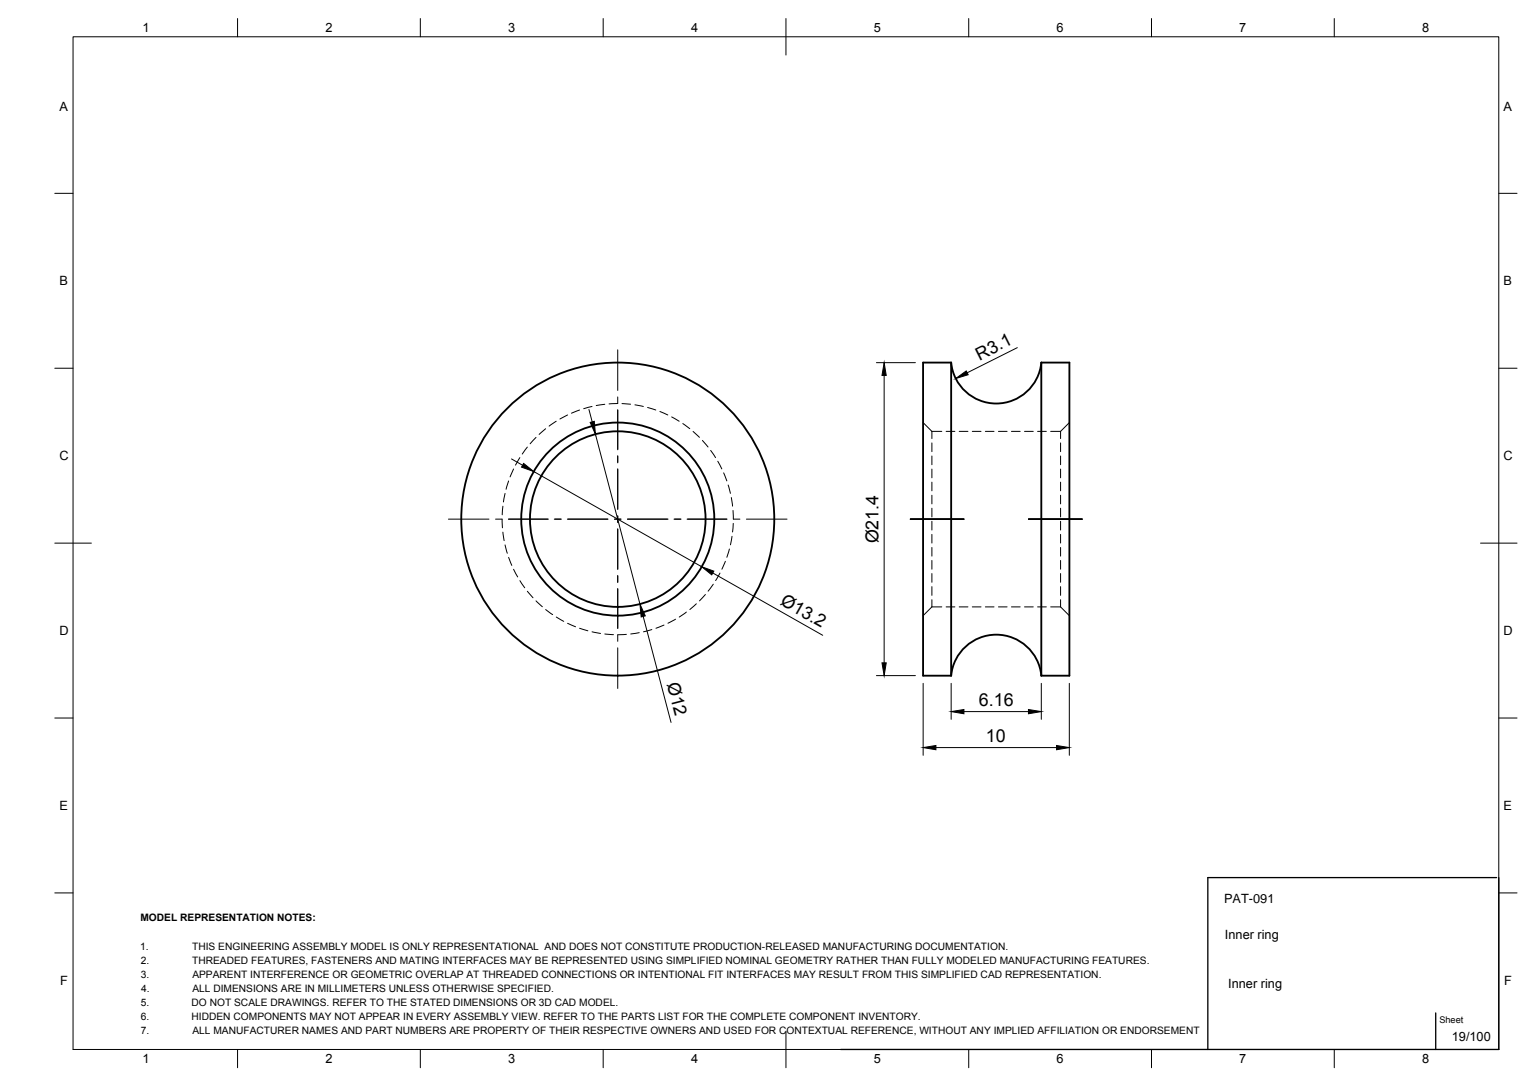
ISO-10303-21;
HEADER;
/* Generated by software containing ST-Developer
 * from STEP Tools, Inc. (www.steptools.com) 
 */

FILE_DESCRIPTION(
/* description */ ('PAT-091'),
/* implementation_level */ '2;1');

FILE_NAME(
/* name */ 'Inner ring.step',
/* time_stamp */ '2026-10-27T15:34:44-07:00',
/* author */ (''),
/* organization */ (''),
/* preprocessor_version */ 'ST-DEVELOPER v20.2',
/* originating_system */ 'Autodesk Translation Framework v15.17.0.0',
/* authorisation */ '');

FILE_SCHEMA (('AUTOMOTIVE_DESIGN { 1 0 10303 214 3 1 1 }'));
ENDSEC;

DATA;
#10=MECHANICAL_DESIGN_GEOMETRIC_PRESENTATION_REPRESENTATION('',(#1070),#25100);
#35=TOROIDAL_SURFACE('',#16134,1.1,0.309556);
#741=CONICAL_SURFACE('',#16145,0.63,0.785398163397448);
#742=CONICAL_SURFACE('',#16152,0.63,0.785398163397448);
#850=SHAPE_REPRESENTATION_RELATIONSHIP('SRR','None',#25618,#960);
#960=ADVANCED_BREP_SHAPE_REPRESENTATION('',(#1191),#25088);
#1070=STYLED_ITEM('',(#26191),#1191);
#1191=MANIFOLD_SOLID_BREP('Body1',#13350);
#1617=FACE_BOUND('',#4000,.T.);
#1618=FACE_BOUND('',#4003,.T.);
#2024=PLANE('',#16147);
#2025=PLANE('',#16150);
#2775=FACE_OUTER_BOUND('',#3995,.T.);
#2776=FACE_OUTER_BOUND('',#3996,.T.);
#2777=FACE_OUTER_BOUND('',#3997,.T.);
#2778=FACE_OUTER_BOUND('',#3998,.T.);
#2779=FACE_OUTER_BOUND('',#3999,.T.);
#2780=FACE_OUTER_BOUND('',#4001,.T.);
#2781=FACE_OUTER_BOUND('',#4002,.T.);
#2782=FACE_OUTER_BOUND('',#4004,.T.);
#3995=EDGE_LOOP('',(#11708,#11709,#11710,#11711,#11712,#11713));
#3996=EDGE_LOOP('',(#11714,#11715,#11716,#11717,#11718));
#3997=EDGE_LOOP('',(#11719,#11720,#11721,#11722));
#3998=EDGE_LOOP('',(#11723,#11724,#11725,#11726));
#3999=EDGE_LOOP('',(#11727));
#4000=EDGE_LOOP('',(#11728));
#4001=EDGE_LOOP('',(#11729,#11730,#11731,#11732,#11733));
#4002=EDGE_LOOP('',(#11734));
#4003=EDGE_LOOP('',(#11735));
#4004=EDGE_LOOP('',(#11736,#11737,#11738,#11739));
#4834=LINE('',#24209,#5574);
#4835=LINE('',#24215,#5575);
#4836=LINE('',#24219,#5576);
#4837=LINE('',#24225,#5577);
#4838=LINE('',#24230,#5578);
#5574=VECTOR('',#20290,1.070235);
#5575=VECTOR('',#20297,0.6);
#5576=VECTOR('',#20302,0.63);
#5577=VECTOR('',#20311,1.070235);
#5578=VECTOR('',#20318,0.63);
#6258=CIRCLE('',#16135,1.070235);
#6259=CIRCLE('',#16136,1.070235);
#6260=CIRCLE('',#16137,0.309556);
#6261=CIRCLE('',#16138,1.070235);
#6262=CIRCLE('',#16139,1.070235);
#6263=CIRCLE('',#16141,1.070235);
#6264=CIRCLE('',#16143,0.6);
#6265=CIRCLE('',#16144,0.6);
#6266=CIRCLE('',#16146,0.66);
#6267=CIRCLE('',#16149,1.070235);
#6268=CIRCLE('',#16151,0.66);
#7291=VERTEX_POINT('',#24198);
#7292=VERTEX_POINT('',#24199);
#7293=VERTEX_POINT('',#24202);
#7294=VERTEX_POINT('',#24204);
#7295=VERTEX_POINT('',#24208);
#7296=VERTEX_POINT('',#24212);
#7297=VERTEX_POINT('',#24214);
#7298=VERTEX_POINT('',#24218);
#7299=VERTEX_POINT('',#24223);
#7300=VERTEX_POINT('',#24227);
#8789=EDGE_CURVE('',#7291,#7292,#6258,.T.);
#8790=EDGE_CURVE('',#7292,#7291,#6259,.T.);
#8791=EDGE_CURVE('',#7292,#7293,#6260,.T.);
#8792=EDGE_CURVE('',#7294,#7293,#6261,.T.);
#8793=EDGE_CURVE('',#7293,#7294,#6262,.T.);
#8794=EDGE_CURVE('',#7294,#7295,#4834,.T.);
#8795=EDGE_CURVE('',#7295,#7295,#6263,.T.);
#8796=EDGE_CURVE('',#7296,#7296,#6264,.T.);
#8797=EDGE_CURVE('',#7296,#7297,#4835,.T.);
#8798=EDGE_CURVE('',#7297,#7297,#6265,.T.);
#8799=EDGE_CURVE('',#7297,#7298,#4836,.T.);
#8800=EDGE_CURVE('',#7298,#7298,#6266,.T.);
#8801=EDGE_CURVE('',#7299,#7299,#6267,.T.);
#8802=EDGE_CURVE('',#7299,#7291,#4837,.T.);
#8803=EDGE_CURVE('',#7300,#7300,#6268,.T.);
#8804=EDGE_CURVE('',#7300,#7296,#4838,.T.);
#11708=ORIENTED_EDGE('',*,*,#8789,.F.);
#11709=ORIENTED_EDGE('',*,*,#8790,.F.);
#11710=ORIENTED_EDGE('',*,*,#8791,.T.);
#11711=ORIENTED_EDGE('',*,*,#8792,.F.);
#11712=ORIENTED_EDGE('',*,*,#8793,.F.);
#11713=ORIENTED_EDGE('',*,*,#8791,.F.);
#11714=ORIENTED_EDGE('',*,*,#8792,.T.);
#11715=ORIENTED_EDGE('',*,*,#8793,.T.);
#11716=ORIENTED_EDGE('',*,*,#8794,.T.);
#11717=ORIENTED_EDGE('',*,*,#8795,.T.);
#11718=ORIENTED_EDGE('',*,*,#8794,.F.);
#11719=ORIENTED_EDGE('',*,*,#8796,.T.);
#11720=ORIENTED_EDGE('',*,*,#8797,.T.);
#11721=ORIENTED_EDGE('',*,*,#8798,.F.);
#11722=ORIENTED_EDGE('',*,*,#8797,.F.);
#11723=ORIENTED_EDGE('',*,*,#8798,.T.);
#11724=ORIENTED_EDGE('',*,*,#8799,.T.);
#11725=ORIENTED_EDGE('',*,*,#8800,.F.);
#11726=ORIENTED_EDGE('',*,*,#8799,.F.);
#11727=ORIENTED_EDGE('',*,*,#8795,.F.);
#11728=ORIENTED_EDGE('',*,*,#8800,.T.);
#11729=ORIENTED_EDGE('',*,*,#8801,.F.);
#11730=ORIENTED_EDGE('',*,*,#8802,.T.);
#11731=ORIENTED_EDGE('',*,*,#8789,.T.);
#11732=ORIENTED_EDGE('',*,*,#8790,.T.);
#11733=ORIENTED_EDGE('',*,*,#8802,.F.);
#11734=ORIENTED_EDGE('',*,*,#8801,.T.);
#11735=ORIENTED_EDGE('',*,*,#8803,.F.);
#11736=ORIENTED_EDGE('',*,*,#8803,.T.);
#11737=ORIENTED_EDGE('',*,*,#8804,.T.);
#11738=ORIENTED_EDGE('',*,*,#8796,.F.);
#11739=ORIENTED_EDGE('',*,*,#8804,.F.);
#12390=CYLINDRICAL_SURFACE('',#16140,1.070235);
#12391=CYLINDRICAL_SURFACE('',#16142,0.6);
#12392=CYLINDRICAL_SURFACE('',#16148,1.070235);
#13142=ADVANCED_FACE('',(#2775),#35,.F.);
#13143=ADVANCED_FACE('',(#2776),#12390,.T.);
#13144=ADVANCED_FACE('',(#2777),#12391,.F.);
#13145=ADVANCED_FACE('',(#2778),#741,.F.);
#13146=ADVANCED_FACE('',(#2779,#1617),#2024,.T.);
#13147=ADVANCED_FACE('',(#2780),#12392,.T.);
#13148=ADVANCED_FACE('',(#2781,#1618),#2025,.T.);
#13149=ADVANCED_FACE('',(#2782),#742,.F.);
#13350=CLOSED_SHELL('',(#13142,#13143,#13144,#13145,#13146,#13147,#13148,
#13149));
#16133=AXIS2_PLACEMENT_3D('',#24196,#20274,#20275);
#16134=AXIS2_PLACEMENT_3D('',#24197,#20276,#20277);
#16135=AXIS2_PLACEMENT_3D('',#24200,#20278,#20279);
#16136=AXIS2_PLACEMENT_3D('',#24201,#20280,#20281);
#16137=AXIS2_PLACEMENT_3D('',#24203,#20282,#20283);
#16138=AXIS2_PLACEMENT_3D('',#24205,#20284,#20285);
#16139=AXIS2_PLACEMENT_3D('',#24206,#20286,#20287);
#16140=AXIS2_PLACEMENT_3D('',#24207,#20288,#20289);
#16141=AXIS2_PLACEMENT_3D('',#24210,#20291,#20292);
#16142=AXIS2_PLACEMENT_3D('',#24211,#20293,#20294);
#16143=AXIS2_PLACEMENT_3D('',#24213,#20295,#20296);
#16144=AXIS2_PLACEMENT_3D('',#24216,#20298,#20299);
#16145=AXIS2_PLACEMENT_3D('',#24217,#20300,#20301);
#16146=AXIS2_PLACEMENT_3D('',#24220,#20303,#20304);
#16147=AXIS2_PLACEMENT_3D('',#24221,#20305,#20306);
#16148=AXIS2_PLACEMENT_3D('',#24222,#20307,#20308);
#16149=AXIS2_PLACEMENT_3D('',#24224,#20309,#20310);
#16150=AXIS2_PLACEMENT_3D('',#24226,#20312,#20313);
#16151=AXIS2_PLACEMENT_3D('',#24228,#20314,#20315);
#16152=AXIS2_PLACEMENT_3D('',#24229,#20316,#20317);
#20274=DIRECTION('axis',(0.,0.,1.));
#20275=DIRECTION('refdir',(1.,0.,0.));
#20276=DIRECTION('center_axis',(0.,-1.,0.));
#20277=DIRECTION('ref_axis',(0.,0.,-1.));
#20278=DIRECTION('center_axis',(0.,-1.,0.));
#20279=DIRECTION('ref_axis',(1.,0.,0.));
#20280=DIRECTION('center_axis',(0.,-1.,0.));
#20281=DIRECTION('ref_axis',(1.,0.,0.));
#20282=DIRECTION('center_axis',(1.,0.,1.22464679914735E-16));
#20283=DIRECTION('ref_axis',(-1.22464679914735E-16,0.,1.));
#20284=DIRECTION('center_axis',(0.,1.,0.));
#20285=DIRECTION('ref_axis',(1.,0.,0.));
#20286=DIRECTION('center_axis',(0.,1.,0.));
#20287=DIRECTION('ref_axis',(1.,0.,0.));
#20288=DIRECTION('center_axis',(0.,-1.,0.));
#20289=DIRECTION('ref_axis',(1.,0.,0.));
#20290=DIRECTION('',(0.,1.,0.));
#20291=DIRECTION('center_axis',(0.,-1.,0.));
#20292=DIRECTION('ref_axis',(1.,0.,0.));
#20293=DIRECTION('center_axis',(0.,-1.,0.));
#20294=DIRECTION('ref_axis',(1.,0.,0.));
#20295=DIRECTION('center_axis',(0.,-1.,0.));
#20296=DIRECTION('ref_axis',(1.,0.,0.));
#20297=DIRECTION('',(0.,1.,0.));
#20298=DIRECTION('center_axis',(0.,-1.,0.));
#20299=DIRECTION('ref_axis',(1.,0.,0.));
#20300=DIRECTION('center_axis',(0.,1.,0.));
#20301=DIRECTION('ref_axis',(1.,0.,0.));
#20302=DIRECTION('',(-0.707106781186548,0.707106781186547,-8.65956056235493E-17));
#20303=DIRECTION('center_axis',(0.,-1.,0.));
#20304=DIRECTION('ref_axis',(1.,0.,0.));
#20305=DIRECTION('center_axis',(0.,1.,0.));
#20306=DIRECTION('ref_axis',(0.,0.,1.));
#20307=DIRECTION('center_axis',(0.,-1.,0.));
#20308=DIRECTION('ref_axis',(1.,0.,0.));
#20309=DIRECTION('center_axis',(0.,-1.,0.));
#20310=DIRECTION('ref_axis',(1.,0.,0.));
#20311=DIRECTION('',(0.,1.,0.));
#20312=DIRECTION('center_axis',(0.,-1.,0.));
#20313=DIRECTION('ref_axis',(0.,0.,-1.));
#20314=DIRECTION('center_axis',(0.,-1.,0.));
#20315=DIRECTION('ref_axis',(1.,0.,0.));
#20316=DIRECTION('center_axis',(0.,-1.,0.));
#20317=DIRECTION('ref_axis',(1.,0.,0.));
#20318=DIRECTION('',(0.707106781186548,0.707106781186547,8.65956056235493E-17));
#24196=CARTESIAN_POINT('',(0.,0.,0.));
#24197=CARTESIAN_POINT('Origin',(0.,0.,0.));
#24198=CARTESIAN_POINT('',(-1.070235,-0.308121667383195,-1.31065986708547E-16));
#24199=CARTESIAN_POINT('',(-1.31065986708547E-16,-0.308121667383195,1.070235));
#24200=CARTESIAN_POINT('Origin',(0.,-0.308121667383195,0.));
#24201=CARTESIAN_POINT('Origin',(0.,-0.308121667383195,0.));
#24202=CARTESIAN_POINT('',(-1.31065986708547E-16,0.308121667383195,1.070235));
#24203=CARTESIAN_POINT('Origin',(-1.34711147906209E-16,0.,1.1));
#24204=CARTESIAN_POINT('',(-1.070235,0.308121667383195,1.31065986708547E-16));
#24205=CARTESIAN_POINT('Origin',(0.,0.308121667383195,0.));
#24206=CARTESIAN_POINT('Origin',(0.,0.308121667383195,0.));
#24207=CARTESIAN_POINT('Origin',(0.,0.,0.));
#24208=CARTESIAN_POINT('',(-1.070235,0.5,-1.31065986708547E-16));
#24209=CARTESIAN_POINT('',(-1.070235,0.,-1.31065986708547E-16));
#24210=CARTESIAN_POINT('Origin',(0.,0.5,0.));
#24211=CARTESIAN_POINT('Origin',(0.,0.,0.));
#24212=CARTESIAN_POINT('',(-0.6,-0.44,-7.34788079488412E-17));
#24213=CARTESIAN_POINT('Origin',(0.,-0.44,0.));
#24214=CARTESIAN_POINT('',(-0.6,0.44,-7.34788079488412E-17));
#24215=CARTESIAN_POINT('',(-0.6,0.,-7.34788079488412E-17));
#24216=CARTESIAN_POINT('Origin',(0.,0.44,0.));
#24217=CARTESIAN_POINT('Origin',(0.,0.47,0.));
#24218=CARTESIAN_POINT('',(-0.66,0.5,-8.08266887437253E-17));
#24219=CARTESIAN_POINT('',(-0.63,0.47,-7.71527483462832E-17));
#24220=CARTESIAN_POINT('Origin',(0.,0.5,0.));
#24221=CARTESIAN_POINT('Origin',(1.070235,0.5,0.));
#24222=CARTESIAN_POINT('Origin',(0.,0.,0.));
#24223=CARTESIAN_POINT('',(-1.070235,-0.5,-1.31065986708547E-16));
#24224=CARTESIAN_POINT('Origin',(0.,-0.5,0.));
#24225=CARTESIAN_POINT('',(-1.070235,0.,-1.31065986708547E-16));
#24226=CARTESIAN_POINT('Origin',(0.66,-0.5,0.));
#24227=CARTESIAN_POINT('',(-0.66,-0.5,-8.08266887437253E-17));
#24228=CARTESIAN_POINT('Origin',(0.,-0.5,0.));
#24229=CARTESIAN_POINT('Origin',(0.,-0.47,0.));
#24230=CARTESIAN_POINT('',(-0.63,-0.47,-7.71527483462832E-17));
#24967=UNCERTAINTY_MEASURE_WITH_UNIT(LENGTH_MEASURE(0.001),#25101,
'DISTANCE_ACCURACY_VALUE',
'Maximum model space distance between geometric entities at asserted c
onnectivities');
#24979=UNCERTAINTY_MEASURE_WITH_UNIT(LENGTH_MEASURE(0.001),#25101,
'DISTANCE_ACCURACY_VALUE',
'Maximum model space distance between geometric entities at asserted c
onnectivities');
#25088=(
GEOMETRIC_REPRESENTATION_CONTEXT(3)
GLOBAL_UNCERTAINTY_ASSIGNED_CONTEXT((#24967))
GLOBAL_UNIT_ASSIGNED_CONTEXT((#25101,#25103,#25104))
REPRESENTATION_CONTEXT('','3D')
);
#25100=(
GEOMETRIC_REPRESENTATION_CONTEXT(3)
GLOBAL_UNCERTAINTY_ASSIGNED_CONTEXT((#24979))
GLOBAL_UNIT_ASSIGNED_CONTEXT((#25101,#25103,#25104))
REPRESENTATION_CONTEXT('','3D')
);
#25101=(
LENGTH_UNIT()
NAMED_UNIT(*)
SI_UNIT(.CENTI.,.METRE.)
);
#25103=(
NAMED_UNIT(*)
PLANE_ANGLE_UNIT()
SI_UNIT($,.RADIAN.)
);
#25104=(
NAMED_UNIT(*)
SI_UNIT($,.STERADIAN.)
SOLID_ANGLE_UNIT()
);
#25213=SHAPE_DEFINITION_REPRESENTATION(#25407,#25618);
#25407=PRODUCT_DEFINITION_SHAPE('',$,#25739);
#25618=SHAPE_REPRESENTATION('',(#16133),#25088);
#25630=PRODUCT_DEFINITION_CONTEXT('part definition',#25992,'design');
#25739=PRODUCT_DEFINITION('Inner ring','Inner ring',#25859,#25630);
#25859=PRODUCT_DEFINITION_FORMATION('',$,#26102);
#25992=APPLICATION_CONTEXT(
'Core Data for Automotive Mechanical Design Process');
#25993=PRODUCT_CONTEXT('part definition',#25992,'mechanical');
#26102=PRODUCT('Inner ring','Inner ring','Inner ring',(#25993));
#26185=COLOUR_RGB('Grey',0.48,0.52,0.57);
#26186=FILL_AREA_STYLE_COLOUR('',#26185);
#26187=FILL_AREA_STYLE('',(#26186));
#26188=SURFACE_STYLE_FILL_AREA(#26187);
#26189=SURFACE_SIDE_STYLE('',(#26188));
#26190=SURFACE_STYLE_USAGE(.BOTH.,#26189);
#26191=PRESENTATION_STYLE_ASSIGNMENT((#26190));
ENDSEC;
END-ISO-10303-21;
